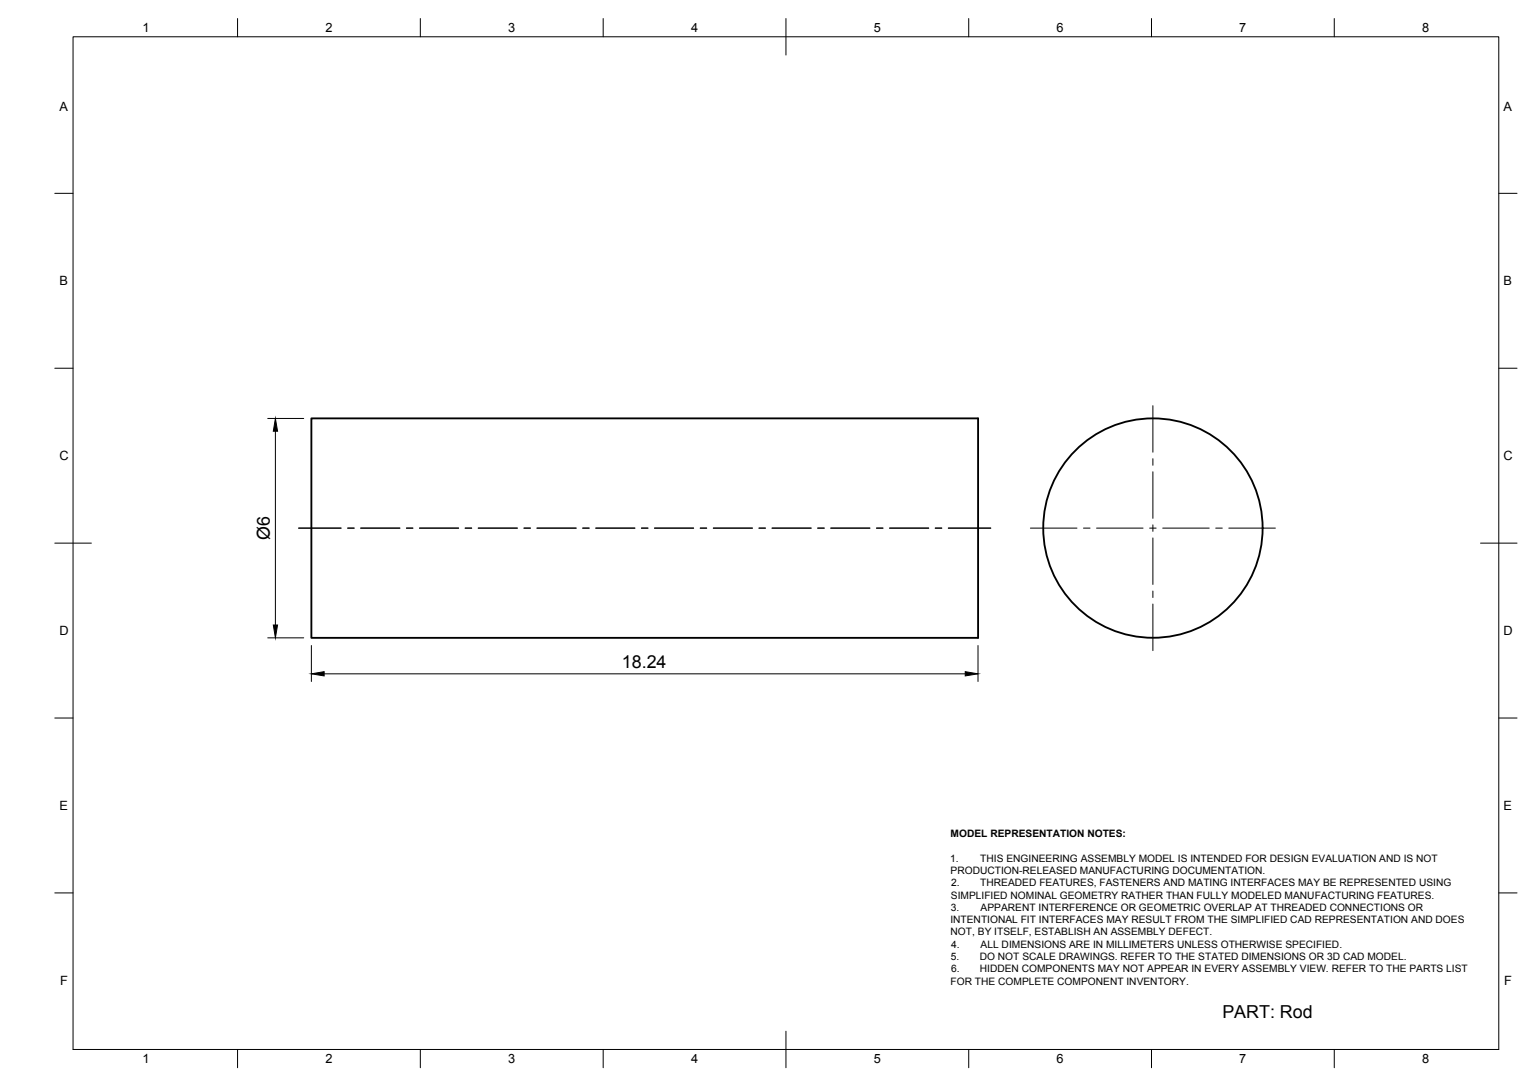
ISO-10303-21;
HEADER;
/* Generated by software containing ST-Developer
 * from STEP Tools, Inc. (www.steptools.com) 
 */

FILE_DESCRIPTION(
/* description */ (''),
/* implementation_level */ '2;1');

FILE_NAME(
/* name */ 'Rod.step',
/* time_stamp */ '2026-10-05T01:33:24-07:00',
/* author */ (''),
/* organization */ (''),
/* preprocessor_version */ 'ST-DEVELOPER v20.2',
/* originating_system */ 'Autodesk Translation Framework v15.15.0.0',
/* authorisation */ '');

FILE_SCHEMA (('AUTOMOTIVE_DESIGN { 1 0 10303 214 3 1 1 }'));
ENDSEC;

DATA;
#10=MECHANICAL_DESIGN_GEOMETRIC_PRESENTATION_REPRESENTATION('',(#82),#1128);
#62=SHAPE_REPRESENTATION_RELATIONSHIP('SRR','None',#1166,#72);
#72=ADVANCED_BREP_SHAPE_REPRESENTATION('',(#92),#1118);
#82=STYLED_ITEM('',(#1225),#92);
#92=MANIFOLD_SOLID_BREP('Body1',#521);
#102=LINE('',#964,#119);
#119=VECTOR('',#753,3.);
#136=CYLINDRICAL_SURFACE('',#646,3.);
#146=FACE_OUTER_BOUND('',#187,.T.);
#147=FACE_OUTER_BOUND('',#188,.T.);
#148=FACE_OUTER_BOUND('',#189,.T.);
#187=EDGE_LOOP('',(#352));
#188=EDGE_LOOP('',(#353,#354,#355,#356));
#189=EDGE_LOOP('',(#357));
#228=CIRCLE('',#645,3.);
#229=CIRCLE('',#647,3.);
#265=VERTEX_POINT('',#959);
#266=VERTEX_POINT('',#962);
#298=EDGE_CURVE('',#265,#265,#228,.T.);
#299=EDGE_CURVE('',#266,#266,#229,.T.);
#300=EDGE_CURVE('',#266,#265,#102,.T.);
#352=ORIENTED_EDGE('',*,*,#298,.F.);
#353=ORIENTED_EDGE('',*,*,#299,.F.);
#354=ORIENTED_EDGE('',*,*,#300,.T.);
#355=ORIENTED_EDGE('',*,*,#298,.T.);
#356=ORIENTED_EDGE('',*,*,#300,.F.);
#357=ORIENTED_EDGE('',*,*,#299,.T.);
#460=PLANE('',#644);
#461=PLANE('',#648);
#480=ADVANCED_FACE('',(#146),#460,.T.);
#481=ADVANCED_FACE('',(#147),#136,.T.);
#482=ADVANCED_FACE('',(#148),#461,.T.);
#521=CLOSED_SHELL('',(#480,#481,#482));
#643=AXIS2_PLACEMENT_3D('',#957,#743,#744);
#644=AXIS2_PLACEMENT_3D('',#958,#745,#746);
#645=AXIS2_PLACEMENT_3D('',#960,#747,#748);
#646=AXIS2_PLACEMENT_3D('',#961,#749,#750);
#647=AXIS2_PLACEMENT_3D('',#963,#751,#752);
#648=AXIS2_PLACEMENT_3D('',#965,#754,#755);
#743=DIRECTION('axis',(0.,0.,1.));
#744=DIRECTION('refdir',(1.,0.,0.));
#745=DIRECTION('center_axis',(-1.,0.,0.));
#746=DIRECTION('ref_axis',(0.,0.,1.));
#747=DIRECTION('center_axis',(1.,0.,0.));
#748=DIRECTION('ref_axis',(0.,0.,-1.));
#749=DIRECTION('center_axis',(1.,0.,0.));
#750=DIRECTION('ref_axis',(0.,0.,-1.));
#751=DIRECTION('center_axis',(1.,0.,0.));
#752=DIRECTION('ref_axis',(0.,0.,-1.));
#753=DIRECTION('',(-1.,0.,0.));
#754=DIRECTION('center_axis',(1.,0.,0.));
#755=DIRECTION('ref_axis',(0.,0.,-1.));
#957=CARTESIAN_POINT('',(0.,0.,0.));
#958=CARTESIAN_POINT('Origin',(0.,0.,-3.));
#959=CARTESIAN_POINT('',(0.,-3.67394039744206E-16,3.));
#960=CARTESIAN_POINT('Origin',(0.,0.,0.));
#961=CARTESIAN_POINT('Origin',(9.11772158674436,0.,0.));
#962=CARTESIAN_POINT('',(18.2354431734887,-3.67394039744206E-16,3.));
#963=CARTESIAN_POINT('Origin',(18.2354431734887,0.,0.));
#964=CARTESIAN_POINT('',(9.11772158674436,-3.67394039744206E-16,3.));
#965=CARTESIAN_POINT('Origin',(18.2354431734887,0.,0.));
#1106=UNCERTAINTY_MEASURE_WITH_UNIT(LENGTH_MEASURE(0.01),#1129,
'DISTANCE_ACCURACY_VALUE',
'Maximum model space distance between geometric entities at asserted c
onnectivities');
#1116=UNCERTAINTY_MEASURE_WITH_UNIT(LENGTH_MEASURE(0.01),#1129,
'DISTANCE_ACCURACY_VALUE',
'Maximum model space distance between geometric entities at asserted c
onnectivities');
#1118=(
GEOMETRIC_REPRESENTATION_CONTEXT(3)
GLOBAL_UNCERTAINTY_ASSIGNED_CONTEXT((#1106))
GLOBAL_UNIT_ASSIGNED_CONTEXT((#1129,#1131,#1132))
REPRESENTATION_CONTEXT('','3D')
);
#1128=(
GEOMETRIC_REPRESENTATION_CONTEXT(3)
GLOBAL_UNCERTAINTY_ASSIGNED_CONTEXT((#1116))
GLOBAL_UNIT_ASSIGNED_CONTEXT((#1129,#1131,#1132))
REPRESENTATION_CONTEXT('','3D')
);
#1129=(
LENGTH_UNIT()
NAMED_UNIT(*)
SI_UNIT(.MILLI.,.METRE.)
);
#1131=(
NAMED_UNIT(*)
PLANE_ANGLE_UNIT()
SI_UNIT($,.RADIAN.)
);
#1132=(
NAMED_UNIT(*)
SI_UNIT($,.STERADIAN.)
SOLID_ANGLE_UNIT()
);
#1134=SHAPE_DEFINITION_REPRESENTATION(#1145,#1166);
#1145=PRODUCT_DEFINITION_SHAPE('',$,#1178);
#1166=SHAPE_REPRESENTATION('',(#643),#1118);
#1176=PRODUCT_DEFINITION_CONTEXT('part definition',#1211,'design');
#1178=PRODUCT_DEFINITION('Rod','Rod',#1189,#1176);
#1189=PRODUCT_DEFINITION_FORMATION('',$,#1214);
#1211=APPLICATION_CONTEXT(
'Core Data for Automotive Mechanical Design Process');
#1212=PRODUCT_CONTEXT('part definition',#1211,'mechanical');
#1214=PRODUCT('Rod','Rod',$,(#1212));
#1225=PRESENTATION_STYLE_ASSIGNMENT((#1229));
#1229=SURFACE_STYLE_USAGE(.BOTH.,#1233);
#1233=SURFACE_SIDE_STYLE('',(#1237));
#1237=SURFACE_STYLE_FILL_AREA(#1241);
#1241=FILL_AREA_STYLE('Opaque(201,201,201)',(#1245));
#1245=FILL_AREA_STYLE_COLOUR('Opaque(201,201,201)',#1249);
#1249=COLOUR_RGB('Opaque(201,201,201)', 0.09019608, 0.27058824, 0.51372549);
ENDSEC;
END-ISO-10303-21;
